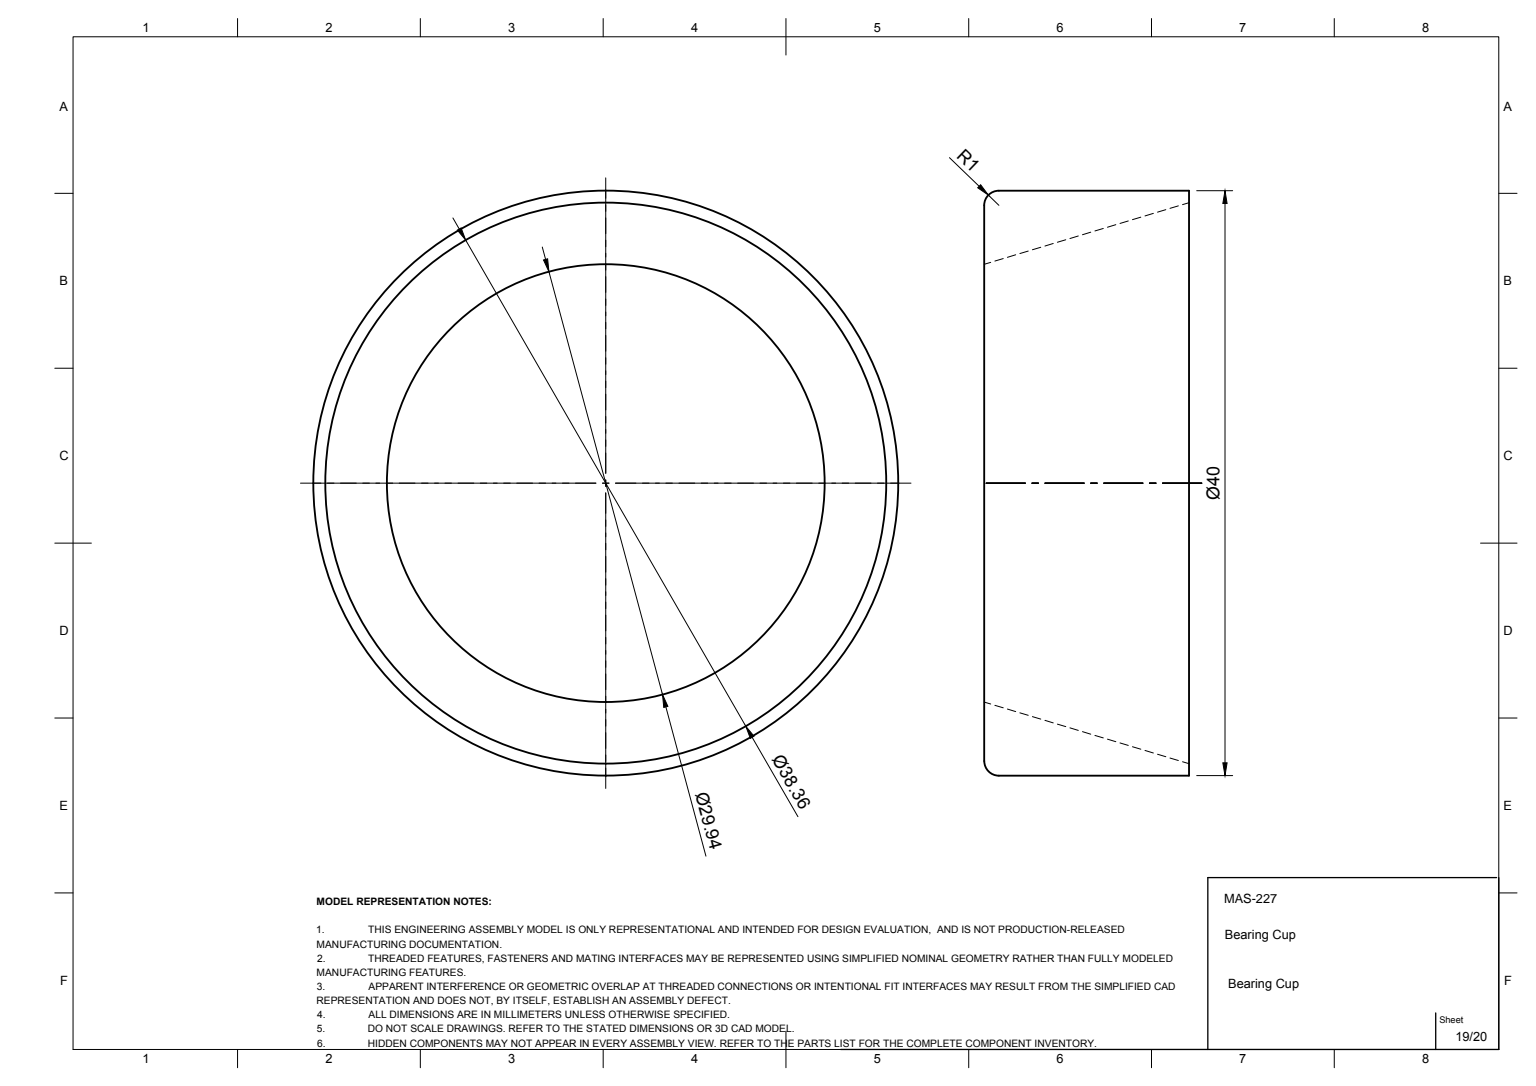
ISO-10303-21;
HEADER;
FILE_DESCRIPTION (('STEP AP214'),
    '1' );
FILE_NAME ( 'Bearing Cup.step', '2026-10-06T08:24:41', ( '' ), ( '' ), 'STEP AP214', 'Unspecified', '' );
FILE_SCHEMA (( 'AUTOMOTIVE_DESIGN' ));
ENDSEC;
DATA;
#4=EDGE_LOOP ( 'NONE', ( #17805, #23711 ) ) ;
#234=AXIS2_PLACEMENT_3D ( 'NONE', #13814, #26508, #13665 ) ;
#321=VECTOR ( 'NONE', #12149, 39.37007874015748143 ) ;
#541=DIRECTION ( 'NONE',  ( 1.000000000000000000, 0.000000000000000000, 0.000000000000000000 ) ) ;
#904=( CONVERSION_BASED_UNIT ( 'INCH', #18242 ) LENGTH_UNIT ( ) NAMED_UNIT ( #24418 ) ) ;
#1032=ADVANCED_FACE ( 'NONE', ( #22429 ), #17495, .T. ) ;
#1033=EDGE_CURVE ( 'NONE', #17335, #10511, #12376, .T. ) ;
#1266=CARTESIAN_POINT ( 'NONE',  ( 0.6791338582677166613, 0.000000000000000000, 0.000000000000000000 ) ) ;
#1363=CARTESIAN_POINT ( 'NONE',  ( 0.1279527559055118058, 0.000000000000000000, 0.000000000000000000 ) ) ;
#1418=DIRECTION ( 'NONE',  ( 0.000000000000000000, 1.000000000000000000, 0.000000000000000000 ) ) ;
#1769=ADVANCED_FACE ( 'NONE', ( #16289 ), #13777, .F. ) ;
#1797=( LENGTH_UNIT ( ) NAMED_UNIT ( * ) SI_UNIT ( $, .METRE. ) ) ;
#1883=DIRECTION ( 'NONE',  ( 1.000000000000000000, 0.000000000000000000, 0.000000000000000000 ) ) ;
#2250=AXIS2_PLACEMENT_3D ( 'NONE', #1266, #16241, #9871 ) ;
#2329=DIRECTION ( 'NONE',  ( -0.9575713609010866323, 0.2881962678142118706, 0.000000000000000000 ) ) ;
#2474=CARTESIAN_POINT ( 'NONE',  ( 0.4035433070866141780, -0.7874015748031496509, 9.642888182262624280E-17 ) ) ;
#2724=STYLED_ITEM ( 'NONE', ( #17058 ), #12201 ) ;
#2735=CARTESIAN_POINT ( 'NONE',  ( 0.2705157149885996093, 0.7122990885670630323, 0.000000000000000000 ) ) ;
#2865=DIRECTION ( 'NONE',  ( 1.000000000000000000, 0.000000000000000000, 0.000000000000000000 ) ) ;
#2930=DIRECTION ( 'NONE',  ( 0.000000000000000000, 1.000000000000000000, 0.000000000000000000 ) ) ;
#3496=( GEOMETRIC_REPRESENTATION_CONTEXT ( 3 ) GLOBAL_UNCERTAINTY_ASSIGNED_CONTEXT ( ( #12494 ) ) GLOBAL_UNIT_ASSIGNED_CONTEXT ( ( #904, #22221, #26589 ) ) REPRESENTATION_CONTEXT ( 'NONE', 'WORKASPACE' ) ) ;
#3623=SURFACE_SIDE_STYLE ('',( #3917 ) ) ;
#3664=ORIENTED_EDGE ( 'NONE', *, *, #25024, .T. ) ;
#3669=CYLINDRICAL_SURFACE ( 'NONE', #14846, 0.7874015748031496509 ) ;
#3840=DIRECTION ( 'NONE',  ( 1.000000000000000000, 0.000000000000000000, 0.000000000000000000 ) ) ;
#3917=SURFACE_STYLE_FILL_AREA ( #27659 ) ;
#3958=EDGE_CURVE ( 'NONE', #8887, #18279, #12135, .T. ) ;
#4056=DIRECTION ( 'NONE',  ( 0.000000000000000000, 1.000000000000000000, 0.000000000000000000 ) ) ;
#4064=( NAMED_UNIT ( * ) PLANE_ANGLE_UNIT ( ) SI_UNIT ( $, .RADIAN. ) ) ;
#4104=ORIENTED_EDGE ( 'NONE', *, *, #24635, .T. ) ;
#4108=MECHANICAL_DESIGN_GEOMETRIC_PRESENTATION_REPRESENTATION('',(#2724),#11773);
#4118=CARTESIAN_POINT ( 'NONE',  ( 0.1279527559055118058, -0.7552056691248124620, -9.248602053916366447E-17 ) ) ;
#4147=DIRECTION ( 'NONE',  ( 0.000000000000000000, 1.000000000000000000, 0.000000000000000000 ) ) ;
#4215=EDGE_LOOP ( 'NONE', ( #10322, #12442 ) ) ;
#4549=ORIENTED_EDGE ( 'NONE', *, *, #1033, .F. ) ;
#4605=VERTEX_POINT ( 'NONE', #20234 ) ;
#4693=ORIENTED_EDGE ( 'NONE', *, *, #25354, .F. ) ;
#4728=LINE ( 'NONE', #2474, #26272 ) ;
#4777=DIRECTION ( 'NONE',  ( 0.000000000000000000, -1.000000000000000000, 0.000000000000000000 ) ) ;
#4794=CARTESIAN_POINT ( 'NONE',  ( 0.1279527559055118058, 0.7874015748031496509, 0.000000000000000000 ) ) ;
#4923=CARTESIAN_POINT ( 'NONE',  ( 0.2705157149885996093, 0.000000000000000000, 0.000000000000000000 ) ) ;
#4982=CARTESIAN_POINT ( 'NONE',  ( 0.1279527559055118058, 0.000000000000000000, 0.000000000000000000 ) ) ;
#5052=CARTESIAN_POINT ( 'NONE',  ( 0.6397637795275591399, 0.000000000000000000, 0.000000000000000000 ) ) ;
#5103=DIRECTION ( 'NONE',  ( 1.000000000000000000, 0.000000000000000000, 0.000000000000000000 ) ) ;
#5173=DIRECTION ( 'NONE',  ( 0.000000000000000000, -1.000000000000000000, 0.000000000000000000 ) ) ;
#5946=DIRECTION ( 'NONE',  ( 0.000000000000000000, 0.000000000000000000, 1.000000000000000000 ) ) ;
#5954=LINE ( 'NONE', #7786, #321 ) ;
#6022=ORIENTED_EDGE ( 'NONE', *, *, #25024, .F. ) ;
#6204=CARTESIAN_POINT ( 'NONE',  ( 0.6397637795275591399, 0.000000000000000000, -0.7874015748031496509 ) ) ;
#6207=ADVANCED_FACE ( 'NONE', ( #20515, #19089 ), #15019, .T. ) ;
#6606=EDGE_LOOP ( 'NONE', ( #3664, #15676, #23156, #25583, #4104 ) ) ;
#6722=CIRCLE ( 'NONE', #16664, 0.7874015748031496509 ) ;
#6755=ORIENTED_EDGE ( 'NONE', *, *, #3958, .F. ) ;
#6809=EDGE_CURVE ( 'NONE', #14040, #13062, #15370, .T. ) ;
#6923=FACE_OUTER_BOUND ( 'NONE', #21322, .T. ) ;
#7041=DIRECTION ( 'NONE',  ( 0.000000000000000000, 1.000000000000000000, 0.000000000000000000 ) ) ;
#7411=CIRCLE ( 'NONE', #27268, 0.7874015748031496509 ) ;
#7425=ORIENTED_EDGE ( 'NONE', *, *, #24446, .F. ) ;
#7542=DIRECTION ( 'NONE',  ( 0.000000000000000000, 1.000000000000000000, 0.000000000000000000 ) ) ;
#7554=PRODUCT_CONTEXT ( 'NONE', #24400, 'mechanical' ) ;
#7729=AXIS2_PLACEMENT_3D ( 'NONE', #19711, #26198, #13469 ) ;
#7786=CARTESIAN_POINT ( 'NONE',  ( 0.4035433070866141780, 0.7874015748031496509, 0.000000000000000000 ) ) ;
#7813=DIRECTION ( 'NONE',  ( 0.000000000000000000, 1.000000000000000000, 0.000000000000000000 ) ) ;
#7937=EDGE_CURVE ( 'NONE', #15244, #14040, #16294, .T. ) ;
#7949=EDGE_CURVE ( 'NONE', #23447, #21391, #19897, .T. ) ;
#8152=DIRECTION ( 'NONE',  ( 0.000000000000000000, 1.000000000000000000, 0.000000000000000000 ) ) ;
#8299=ORIENTED_EDGE ( 'NONE', *, *, #24446, .T. ) ;
#8436=( NAMED_UNIT ( * ) SI_UNIT ( $, .STERADIAN. ) SOLID_ANGLE_UNIT ( ) ) ;
#8887=VERTEX_POINT ( 'NONE', #4118 ) ;
#8990=EDGE_LOOP ( 'NONE', ( #9299, #26916, #9353, #15904, #4549 ) ) ;
#9271=DIRECTION ( 'NONE',  ( 1.000000000000000000, 0.000000000000000000, 0.000000000000000000 ) ) ;
#9299=ORIENTED_EDGE ( 'NONE', *, *, #13201, .F. ) ;
#9353=ORIENTED_EDGE ( 'NONE', *, *, #26644, .T. ) ;
#9452=ADVANCED_FACE ( 'NONE', ( #20546, #20260 ), #22238, .T. ) ;
#9491=AXIS2_PLACEMENT_3D ( 'NONE', #10074, #14050, #7542 ) ;
#9505=DIRECTION ( 'NONE',  ( 0.000000000000000000, 1.000000000000000000, 0.000000000000000000 ) ) ;
#9871=DIRECTION ( 'NONE',  ( 0.000000000000000000, -1.000000000000000000, 0.000000000000000000 ) ) ;
#9895=CARTESIAN_POINT ( 'NONE',  ( 0.4035433070866141780, 0.000000000000000000, 0.000000000000000000 ) ) ;
#9975=DIRECTION ( 'NONE',  ( 1.000000000000000000, 0.000000000000000000, 0.000000000000000000 ) ) ;
#10038=CIRCLE ( 'NONE', #17712, 0.5893189861902062843 ) ;
#10074=CARTESIAN_POINT ( 'NONE',  ( 0.1279527559055118058, 0.000000000000000000, 0.000000000000000000 ) ) ;
#10256=VERTEX_POINT ( 'NONE', #22751 ) ;
#10322=ORIENTED_EDGE ( 'NONE', *, *, #22177, .T. ) ;
#10423=ORIENTED_EDGE ( 'NONE', *, *, #22453, .T. ) ;
#10511=VERTEX_POINT ( 'NONE', #6204 ) ;
#10538=CARTESIAN_POINT ( 'NONE',  ( 0.6791338582677166613, 0.000000000000000000, -0.7480314960629921295 ) ) ;
#10650=ORIENTED_EDGE ( 'NONE', *, *, #1033, .T. ) ;
#11072=TOROIDAL_SURFACE ( 'NONE', #18264, 0.7480314960629921295, 0.03937007874015747977 ) ;
#11263=EDGE_CURVE ( 'NONE', #20543, #8887, #26028, .T. ) ;
#11462=CARTESIAN_POINT ( 'NONE',  ( 0.1279527559055118058, -0.7874015748031496509, 9.642888182262624280E-17 ) ) ;
#11510=CIRCLE ( 'NONE', #25966, 0.03937007874015751446 ) ;
#11610=AXIS2_PLACEMENT_3D ( 'NONE', #4982, #24606, #16153 ) ;
#11764=( LENGTH_UNIT ( ) NAMED_UNIT ( * ) SI_UNIT ( $, .METRE. ) ) ;
#11773=( GEOMETRIC_REPRESENTATION_CONTEXT ( 3 ) GLOBAL_UNCERTAINTY_ASSIGNED_CONTEXT ( ( #14129 ) ) GLOBAL_UNIT_ASSIGNED_CONTEXT ( ( #14822, #4064, #8436 ) ) REPRESENTATION_CONTEXT ( 'NONE', 'WORKASPACE' ) ) ;
#11866=VECTOR ( 'NONE', #19533, 39.37007874015748143 ) ;
#11939=CIRCLE ( 'NONE', #18699, 0.7874015748031496509 ) ;
#12135=CIRCLE ( 'NONE', #14879, 0.7552056691767480290 ) ;
#12149=DIRECTION ( 'NONE',  ( 1.000000000000000000, 0.000000000000000000, 0.000000000000000000 ) ) ;
#12179=EDGE_LOOP ( 'NONE', ( #21943, #17068, #27719, #6755 ) ) ;
#12201=MANIFOLD_SOLID_BREP ( 'Bearing Cup', #23648 ) ;
#12299=ORIENTED_EDGE ( 'NONE', *, *, #17135, .T. ) ;
#12376=CIRCLE ( 'NONE', #234, 0.7874015748031496509 ) ;
#12395=SURFACE_STYLE_USAGE ( .BOTH. , #3623 ) ;
#12442=ORIENTED_EDGE ( 'NONE', *, *, #3958, .T. ) ;
#12494=UNCERTAINTY_MEASURE_WITH_UNIT (LENGTH_MEASURE( 1.000000000000000082E-05 ), #904, 'distance_accuracy_value', 'NONE') ;
#12889=DIRECTION ( 'NONE',  ( 1.000000000000000000, 0.000000000000000000, 0.000000000000000000 ) ) ;
#13062=VERTEX_POINT ( 'NONE', #10538 ) ;
#13141=DIRECTION ( 'NONE',  ( 0.000000000000000000, -1.000000000000000000, 0.000000000000000000 ) ) ;
#13163=CARTESIAN_POINT ( 'NONE',  ( 0.6397637795275591399, -0.7874015748031496509, 9.642888182262624280E-17 ) ) ;
#13201=EDGE_CURVE ( 'NONE', #21391, #17335, #4728, .T. ) ;
#13429=FACE_OUTER_BOUND ( 'NONE', #25801, .T. ) ;
#13451=EDGE_CURVE ( 'NONE', #20543, #4605, #10038, .T. ) ;
#13469=DIRECTION ( 'NONE',  ( 0.000000000000000000, 1.224646799147353207E-16, 1.000000000000000000 ) ) ;
#13665=DIRECTION ( 'NONE',  ( 0.000000000000000000, -1.000000000000000000, 0.000000000000000000 ) ) ;
#13728=DIRECTION ( 'NONE',  ( 0.000000000000000000, -1.000000000000000000, 0.000000000000000000 ) ) ;
#13777=CONICAL_SURFACE ( 'NONE', #18735, 0.7122990885670630323, 0.2923426493749994304 ) ;
#13800=DIRECTION ( 'NONE',  ( 1.000000000000000000, 0.000000000000000000, 0.000000000000000000 ) ) ;
#13814=CARTESIAN_POINT ( 'NONE',  ( 0.6397637795275591399, 0.000000000000000000, 0.000000000000000000 ) ) ;
#14040=VERTEX_POINT ( 'NONE', #21037 ) ;
#14050=DIRECTION ( 'NONE',  ( 1.000000000000000000, 0.000000000000000000, 0.000000000000000000 ) ) ;
#14129=UNCERTAINTY_MEASURE_WITH_UNIT (LENGTH_MEASURE( 1.000000000000000082E-05 ), #14822, 'distance_accuracy_value', 'NONE') ;
#14172=CIRCLE ( 'NONE', #17757, 0.7480314960629921295 ) ;
#14392=FILL_AREA_STYLE_COLOUR ( '', #23961 ) ;
#14558=ORIENTED_EDGE ( 'NONE', *, *, #11263, .T. ) ;
#14816=CARTESIAN_POINT ( 'NONE',  ( 0.1279527559055118058, 0.000000000000000000, 0.000000000000000000 ) ) ;
#14822=( CONVERSION_BASED_UNIT ( 'INCH', #18876 ) LENGTH_UNIT ( ) NAMED_UNIT ( #27277 ) ) ;
#14846=AXIS2_PLACEMENT_3D ( 'NONE', #9895, #16263, #1418 ) ;
#14879=AXIS2_PLACEMENT_3D ( 'NONE', #14816, #16917, #4056 ) ;
#15019=PLANE ( 'NONE',  #20708 ) ;
#15171=CARTESIAN_POINT ( 'NONE',  ( 0.2705157149885996093, -0.7122990885670630323, -8.723147988492308551E-17 ) ) ;
#15244=VERTEX_POINT ( 'NONE', #16816 ) ;
#15370=CIRCLE ( 'NONE', #2250, 0.7480314960629921295 ) ;
#15676=ORIENTED_EDGE ( 'NONE', *, *, #7937, .T. ) ;
#15856=CARTESIAN_POINT ( 'NONE',  ( 0.2705157149885996093, 0.000000000000000000, 0.000000000000000000 ) ) ;
#15860=ORIENTED_EDGE ( 'NONE', *, *, #6809, .F. ) ;
#15904=ORIENTED_EDGE ( 'NONE', *, *, #24635, .F. ) ;
#15943=DIRECTION ( 'NONE',  ( -1.000000000000000000, 0.000000000000000000, 0.000000000000000000 ) ) ;
#16068=FACE_OUTER_BOUND ( 'NONE', #6606, .T. ) ;
#16153=DIRECTION ( 'NONE',  ( 0.000000000000000000, 1.000000000000000000, 0.000000000000000000 ) ) ;
#16241=DIRECTION ( 'NONE',  ( -1.000000000000000000, 0.000000000000000000, 0.000000000000000000 ) ) ;
#16242=ADVANCED_FACE ( 'NONE', ( #13429 ), #11072, .T. ) ;
#16263=DIRECTION ( 'NONE',  ( 1.000000000000000000, 0.000000000000000000, 0.000000000000000000 ) ) ;
#16289=FACE_OUTER_BOUND ( 'NONE', #12179, .T. ) ;
#16294=CIRCLE ( 'NONE', #7729, 0.03937007874015751446 ) ;
#16664=AXIS2_PLACEMENT_3D ( 'NONE', #1363, #9975, #8152 ) ;
#16686=AXIS2_PLACEMENT_3D ( 'NONE', #5052, #26255, #4777 ) ;
#16816=CARTESIAN_POINT ( 'NONE',  ( 0.6397637795275591399, 9.642888182262624280E-17, 0.7874015748031496509 ) ) ;
#16862=DIRECTION ( 'NONE',  ( -1.000000000000000000, 0.000000000000000000, 0.000000000000000000 ) ) ;
#16917=DIRECTION ( 'NONE',  ( 1.000000000000000000, 0.000000000000000000, 0.000000000000000000 ) ) ;
#17058=PRESENTATION_STYLE_ASSIGNMENT (( #12395 ) ) ;
#17068=ORIENTED_EDGE ( 'NONE', *, *, #13451, .T. ) ;
#17121=CARTESIAN_POINT ( 'NONE',  ( 0.6791338582677166613, 0.000000000000000000, 0.000000000000000000 ) ) ;
#17135=EDGE_CURVE ( 'NONE', #4605, #20543, #18487, .T. ) ;
#17136=DIRECTION ( 'NONE',  ( 0.000000000000000000, 0.000000000000000000, -1.000000000000000000 ) ) ;
#17335=VERTEX_POINT ( 'NONE', #13163 ) ;
#17495=CYLINDRICAL_SURFACE ( 'NONE', #17786, 0.7874015748031496509 ) ;
#17712=AXIS2_PLACEMENT_3D ( 'NONE', #17121, #3840, #25454 ) ;
#17720=DIRECTION ( 'NONE',  ( 1.000000000000000000, 0.000000000000000000, 0.000000000000000000 ) ) ;
#17757=AXIS2_PLACEMENT_3D ( 'NONE', #20946, #16862, #20805 ) ;
#17766=ORIENTED_EDGE ( 'NONE', *, *, #13201, .T. ) ;
#17786=AXIS2_PLACEMENT_3D ( 'NONE', #23996, #9271, #7041 ) ;
#17805=ORIENTED_EDGE ( 'NONE', *, *, #7949, .F. ) ;
#17906=APPLICATION_CONTEXT ( 'automotive_design' ) ;
#18242=LENGTH_MEASURE_WITH_UNIT ( LENGTH_MEASURE( 0.02539999999999999897 ), #11764 ) ;
#18264=AXIS2_PLACEMENT_3D ( 'NONE', #23785, #12889, #17136 ) ;
#18279=VERTEX_POINT ( 'NONE', #27508 ) ;
#18282=EDGE_CURVE ( 'NONE', #21391, #23447, #6722, .T. ) ;
#18487=CIRCLE ( 'NONE', #19855, 0.5893189861902062843 ) ;
#18699=AXIS2_PLACEMENT_3D ( 'NONE', #24945, #13800, #5173 ) ;
#18735=AXIS2_PLACEMENT_3D ( 'NONE', #15856, #24460, #7813 ) ;
#18876=LENGTH_MEASURE_WITH_UNIT ( LENGTH_MEASURE( 0.02539999999999999897 ), #1797 ) ;
#19059=CARTESIAN_POINT ( 'NONE',  ( 0.1279527559055118058, 0.7713036219899488399, 0.000000000000000000 ) ) ;
#19089=FACE_OUTER_BOUND ( 'NONE', #4, .T. ) ;
#19098=TOROIDAL_SURFACE ( 'NONE', #26312, 0.7480314960629921295, 0.03937007874015747977 ) ;
#19205=DIRECTION ( 'NONE',  ( -1.000000000000000000, 0.000000000000000000, 0.000000000000000000 ) ) ;
#19533=DIRECTION ( 'NONE',  ( -0.9575713609010866323, -0.2881962678142118706, -3.529386369048878649E-17 ) ) ;
#19542=AXIS2_PLACEMENT_3D ( 'NONE', #26894, #2865, #9505 ) ;
#19711=CARTESIAN_POINT ( 'NONE',  ( 0.6397637795275591399, 9.160743773149492203E-17, 0.7480314960629921295 ) ) ;
#19855=AXIS2_PLACEMENT_3D ( 'NONE', #21383, #1883, #4147 ) ;
#19897=CIRCLE ( 'NONE', #9491, 0.7874015748031496509 ) ;
#20046=ORIENTED_EDGE ( 'NONE', *, *, #26644, .F. ) ;
#20234=CARTESIAN_POINT ( 'NONE',  ( 0.6791338582677166613, 0.5893189861902062843, 0.000000000000000000 ) ) ;
#20260=FACE_OUTER_BOUND ( 'NONE', #21590, .T. ) ;
#20403=PRODUCT_DEFINITION_CONTEXT ( 'detailed design', #17906, 'design' ) ;
#20515=FACE_BOUND ( 'NONE', #4215, .T. ) ;
#20528=ADVANCED_FACE ( 'NONE', ( #26997 ), #3669, .T. ) ;
#20543=VERTEX_POINT ( 'NONE', #27419 ) ;
#20546=FACE_BOUND ( 'NONE', #27228, .T. ) ;
#20593=AXIS2_PLACEMENT_3D ( 'NONE', #4923, #15943, #2930 ) ;
#20708=AXIS2_PLACEMENT_3D ( 'NONE', #19059, #19205, #5946 ) ;
#20805=DIRECTION ( 'NONE',  ( 0.000000000000000000, -1.000000000000000000, 0.000000000000000000 ) ) ;
#20946=CARTESIAN_POINT ( 'NONE',  ( 0.6791338582677166613, 0.000000000000000000, 0.000000000000000000 ) ) ;
#21036=CONICAL_SURFACE ( 'NONE', #20593, 0.7122990885670630323, 0.2923426493749994304 ) ;
#21037=CARTESIAN_POINT ( 'NONE',  ( 0.6791338582677166613, 9.401815977706058242E-17, 0.7480314960629921295 ) ) ;
#21322=EDGE_LOOP ( 'NONE', ( #12299, #14558, #26087, #4693 ) ) ;
#21380=ORIENTED_EDGE ( 'NONE', *, *, #22453, .F. ) ;
#21383=CARTESIAN_POINT ( 'NONE',  ( 0.6791338582677166613, 0.000000000000000000, 0.000000000000000000 ) ) ;
#21391=VERTEX_POINT ( 'NONE', #11462 ) ;
#21429=VECTOR ( 'NONE', #2329, 39.37007874015748143 ) ;
#21590=EDGE_LOOP ( 'NONE', ( #7425, #15860 ) ) ;
#21650=CIRCLE ( 'NONE', #16686, 0.7874015748031496509 ) ;
#21701=LINE ( 'NONE', #2735, #21429 ) ;
#21727=ORIENTED_EDGE ( 'NONE', *, *, #7937, .F. ) ;
#21771=CARTESIAN_POINT ( 'NONE',  ( 0.6397637795275591399, 0.000000000000000000, -0.7480314960629921295 ) ) ;
#21943=ORIENTED_EDGE ( 'NONE', *, *, #11263, .F. ) ;
#22177=EDGE_CURVE ( 'NONE', #18279, #8887, #23813, .T. ) ;
#22221=( NAMED_UNIT ( * ) PLANE_ANGLE_UNIT ( ) SI_UNIT ( $, .RADIAN. ) ) ;
#22238=PLANE ( 'NONE',  #19542 ) ;
#22429=FACE_OUTER_BOUND ( 'NONE', #23306, .T. ) ;
#22453=EDGE_CURVE ( 'NONE', #15244, #17335, #21650, .T. ) ;
#22751=CARTESIAN_POINT ( 'NONE',  ( 0.6397637795275591399, 0.7874015748031496509, 0.000000000000000000 ) ) ;
#23156=ORIENTED_EDGE ( 'NONE', *, *, #6809, .T. ) ;
#23306=EDGE_LOOP ( 'NONE', ( #24566, #17766, #21380, #6022, #20046 ) ) ;
#23447=VERTEX_POINT ( 'NONE', #4794 ) ;
#23627=DIRECTION ( 'NONE',  ( 0.000000000000000000, 0.000000000000000000, -1.000000000000000000 ) ) ;
#23648=CLOSED_SHELL ( 'NONE', ( #23870, #1032, #26955, #1769, #6207, #9452, #20528, #16242 ) ) ;
#23711=ORIENTED_EDGE ( 'NONE', *, *, #18282, .F. ) ;
#23722=ORIENTED_EDGE ( 'NONE', *, *, #13451, .F. ) ;
#23777=ORIENTED_EDGE ( 'NONE', *, *, #17135, .F. ) ;
#23785=CARTESIAN_POINT ( 'NONE',  ( 0.6397637795275591399, 0.000000000000000000, 0.000000000000000000 ) ) ;
#23813=CIRCLE ( 'NONE', #11610, 0.7552056691767480290 ) ;
#23854=ORIENTED_EDGE ( 'NONE', *, *, #25622, .T. ) ;
#23870=ADVANCED_FACE ( 'NONE', ( #16068 ), #19098, .T. ) ;
#23961=COLOUR_RGB ( '', 0.66274510, 0.83137255, 0.94901961) ;
#23996=CARTESIAN_POINT ( 'NONE',  ( 0.4035433070866141780, 0.000000000000000000, 0.000000000000000000 ) ) ;
#24257=CARTESIAN_POINT ( 'NONE',  ( 0.6397637795275591399, 0.000000000000000000, 0.000000000000000000 ) ) ;
#24400=APPLICATION_CONTEXT ( 'automotive_design' ) ;
#24418=DIMENSIONAL_EXPONENTS ( 1.000000000000000000, 0.000000000000000000, 0.000000000000000000, 0.000000000000000000, 0.000000000000000000, 0.000000000000000000, 0.000000000000000000 ) ;
#24446=EDGE_CURVE ( 'NONE', #13062, #14040, #14172, .T. ) ;
#24452=CARTESIAN_POINT ( 'NONE',  ( 0.6397637795275591399, 0.000000000000000000, 0.000000000000000000 ) ) ;
#24460=DIRECTION ( 'NONE',  ( -1.000000000000000000, 0.000000000000000000, 0.000000000000000000 ) ) ;
#24566=ORIENTED_EDGE ( 'NONE', *, *, #7949, .T. ) ;
#24606=DIRECTION ( 'NONE',  ( 1.000000000000000000, 0.000000000000000000, 0.000000000000000000 ) ) ;
#24635=EDGE_CURVE ( 'NONE', #10511, #10256, #7411, .T. ) ;
#24945=CARTESIAN_POINT ( 'NONE',  ( 0.6397637795275591399, 0.000000000000000000, 0.000000000000000000 ) ) ;
#25024=EDGE_CURVE ( 'NONE', #10256, #15244, #11939, .T. ) ;
#25354=EDGE_CURVE ( 'NONE', #4605, #18279, #21701, .T. ) ;
#25454=DIRECTION ( 'NONE',  ( 0.000000000000000000, 1.000000000000000000, 0.000000000000000000 ) ) ;
#25583=ORIENTED_EDGE ( 'NONE', *, *, #25622, .F. ) ;
#25622=EDGE_CURVE ( 'NONE', #10511, #13062, #11510, .T. ) ;
#25801=EDGE_LOOP ( 'NONE', ( #21727, #10423, #10650, #23854, #8299 ) ) ;
#25966=AXIS2_PLACEMENT_3D ( 'NONE', #21771, #13141, #23627 ) ;
#26028=LINE ( 'NONE', #15171, #11866 ) ;
#26087=ORIENTED_EDGE ( 'NONE', *, *, #22177, .F. ) ;
#26198=DIRECTION ( 'NONE',  ( 0.000000000000000000, 1.000000000000000000, -1.224646799147353207E-16 ) ) ;
#26243=DIRECTION ( 'NONE',  ( 0.000000000000000000, 0.000000000000000000, -1.000000000000000000 ) ) ;
#26255=DIRECTION ( 'NONE',  ( 1.000000000000000000, 0.000000000000000000, 0.000000000000000000 ) ) ;
#26272=VECTOR ( 'NONE', #17720, 39.37007874015748143 ) ;
#26312=AXIS2_PLACEMENT_3D ( 'NONE', #24257, #541, #26243 ) ;
#26508=DIRECTION ( 'NONE',  ( 1.000000000000000000, 0.000000000000000000, 0.000000000000000000 ) ) ;
#26589=( NAMED_UNIT ( * ) SI_UNIT ( $, .STERADIAN. ) SOLID_ANGLE_UNIT ( ) ) ;
#26644=EDGE_CURVE ( 'NONE', #23447, #10256, #5954, .T. ) ;
#26894=CARTESIAN_POINT ( 'NONE',  ( 0.6791338582677166613, 0.6883602804966771904, 0.000000000000000000 ) ) ;
#26916=ORIENTED_EDGE ( 'NONE', *, *, #18282, .T. ) ;
#26955=ADVANCED_FACE ( 'NONE', ( #6923 ), #21036, .F. ) ;
#26997=FACE_OUTER_BOUND ( 'NONE', #8990, .T. ) ;
#27228=EDGE_LOOP ( 'NONE', ( #23777, #23722 ) ) ;
#27268=AXIS2_PLACEMENT_3D ( 'NONE', #24452, #5103, #13728 ) ;
#27277=DIMENSIONAL_EXPONENTS ( 1.000000000000000000, 0.000000000000000000, 0.000000000000000000, 0.000000000000000000, 0.000000000000000000, 0.000000000000000000, 0.000000000000000000 ) ;
#27419=CARTESIAN_POINT ( 'NONE',  ( 0.6791338582677166613, -0.5893189861902062843, -8.232839077402887083E-17 ) ) ;
#27508=CARTESIAN_POINT ( 'NONE',  ( 0.1279527559055118058, 0.7552056691248124620, 0.000000000000000000 ) ) ;
#27659=FILL_AREA_STYLE ('',( #14392 ) ) ;
#27719=ORIENTED_EDGE ( 'NONE', *, *, #25354, .T. ) ;
#27927=CARTESIAN_POINT ( '', ( 0.0, 0.0, 0.0 ) ) ;
#27928=DIRECTION ( '', ( 0.0, 0.0, 1.0 ) ) ;
#27929=DIRECTION ( '', ( 1.0, 0.0, 0.0 ) ) ;
#27930=AXIS2_PLACEMENT_3D ( '', #27927, #27928, #27929 ) ;
#27931=ADVANCED_BREP_SHAPE_REPRESENTATION ( 'Bearing Cup', ( #12201, #27930, #27941 ), #3496 ) ;
#27932=PRODUCT ( 'Bearing Cup', 'Bearing Cup', '', ( #7554 ) ) ;
#27933=PRODUCT_DEFINITION_FORMATION_WITH_SPECIFIED_SOURCE ( 'ANY', '', #27932, .NOT_KNOWN. ) ;
#27934=PRODUCT_DEFINITION ( 'Bearing Cup', '', #27933, #20403 ) ;
#27935=PRODUCT_DEFINITION_SHAPE ( '', '', #27934 ) ;
#27936=SHAPE_DEFINITION_REPRESENTATION ( #27935, #27931 ) ;
#27938=CARTESIAN_POINT ( '', ( 0.0, 0.0, 0.0 ) ) ;
#27939=DIRECTION ( '', ( 0.0, 0.0, 1.0 ) ) ;
#27940=DIRECTION ( '', ( 1.0, 0.0, 0.0 ) ) ;
#27941=AXIS2_PLACEMENT_3D ( '', #27938, #27939, #27940 ) ;
ENDSEC;
END-ISO-10303-21;
